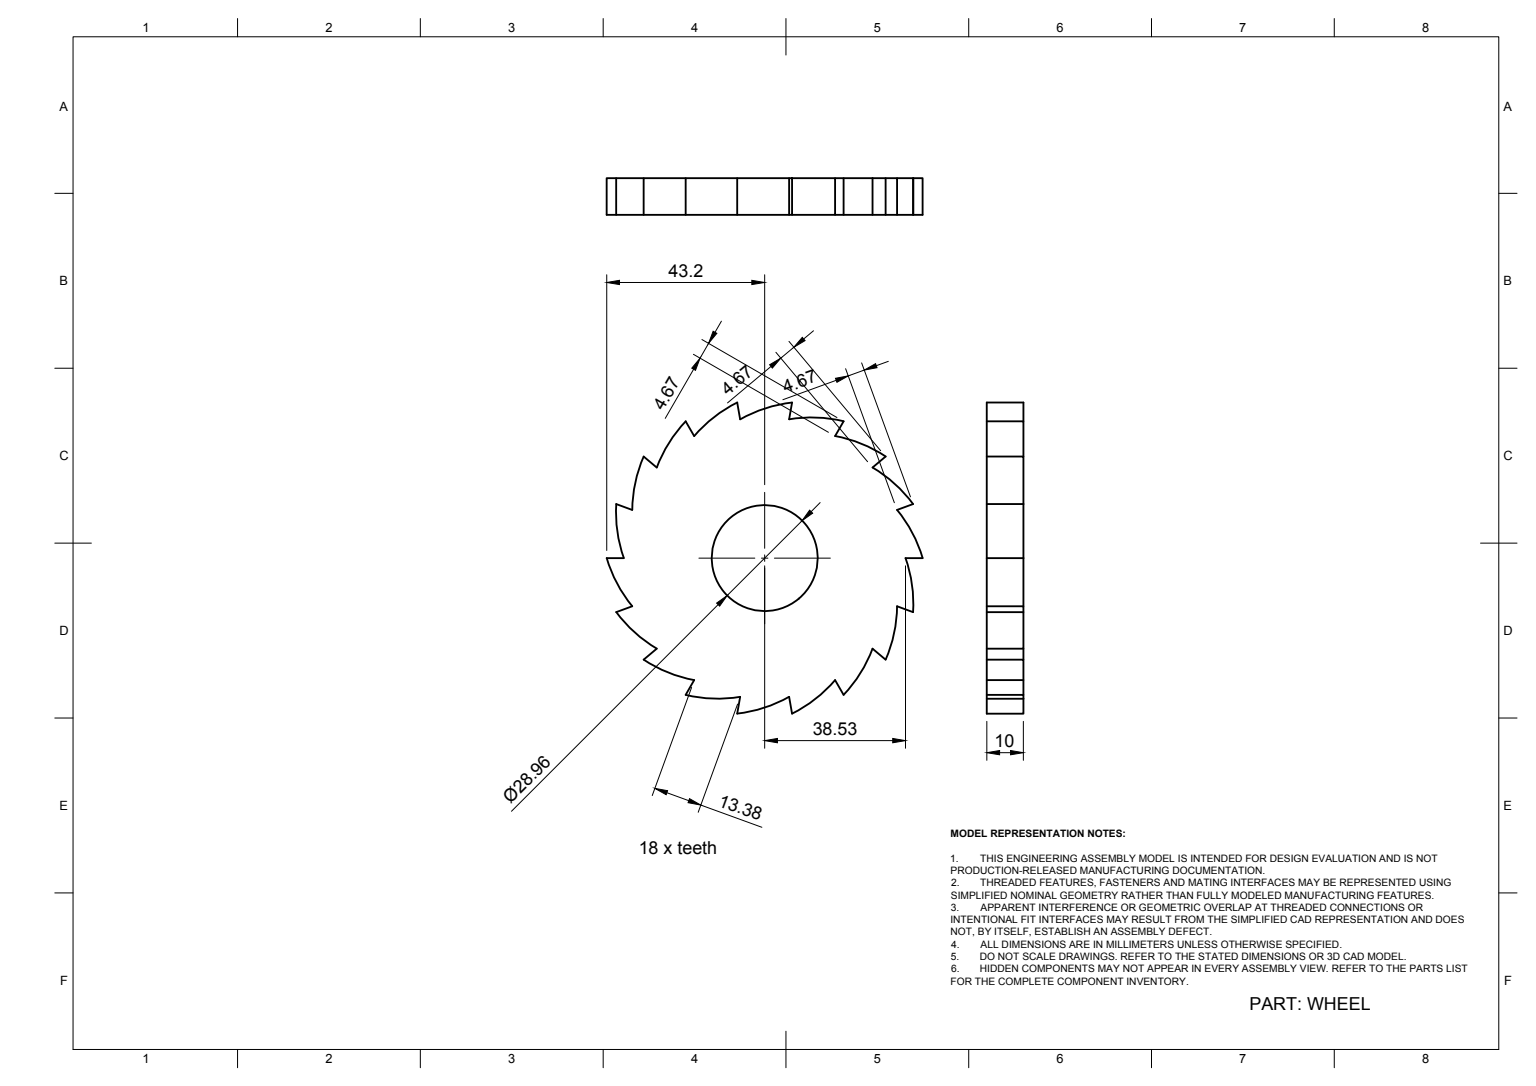
ISO-10303-21;
HEADER;
/* Generated by software containing ST-Developer
 * from STEP Tools, Inc. (www.steptools.com) 
 */

FILE_DESCRIPTION(
/* description */ (''),
/* implementation_level */ '2;1');

FILE_NAME(
/* name */ 'Wheel.step',
/* time_stamp */ '2026-09-20T22:38:01+06:00',
/* author */ (''),
/* organization */ (''),
/* preprocessor_version */ 'ST-DEVELOPER v20.2',
/* originating_system */ 'Autodesk Translation Framework v15.15.0.0',
/* authorisation */ '');

FILE_SCHEMA (('AUTOMOTIVE_DESIGN { 1 0 10303 214 3 1 1 }'));
ENDSEC;

DATA;
#10=MECHANICAL_DESIGN_GEOMETRIC_PRESENTATION_REPRESENTATION('',(#84),#4079);
#68=SHAPE_REPRESENTATION_RELATIONSHIP('SRR','None',#4111,#76);
#76=ADVANCED_BREP_SHAPE_REPRESENTATION('',(#92),#4071);
#84=STYLED_ITEM('',(#4160),#92);
#92=MANIFOLD_SOLID_BREP('Wheel',#1443);
#100=FACE_BOUND('',#285,.T.);
#101=FACE_BOUND('',#308,.T.);
#106=CIRCLE('',#1544,37.4987147312734);
#107=CIRCLE('',#1545,37.4987147312734);
#108=CIRCLE('',#1548,37.4987147312734);
#109=CIRCLE('',#1549,37.4987147312734);
#110=CIRCLE('',#1550,37.4987147312734);
#111=CIRCLE('',#1551,37.4987147312734);
#112=CIRCLE('',#1552,37.4987147312734);
#113=CIRCLE('',#1553,37.4987147312734);
#114=CIRCLE('',#1554,37.4987147312734);
#115=CIRCLE('',#1555,37.4987147312735);
#116=CIRCLE('',#1556,37.4987147312734);
#117=CIRCLE('',#1557,37.4987147312734);
#118=CIRCLE('',#1558,37.4987147312734);
#119=CIRCLE('',#1559,37.4987147312734);
#120=CIRCLE('',#1560,37.4987147312734);
#121=CIRCLE('',#1561,37.4987147312734);
#122=CIRCLE('',#1562,37.4987147312734);
#123=CIRCLE('',#1563,37.4987147312734);
#124=CIRCLE('',#1564,37.4987147312734);
#125=CIRCLE('',#1565,14.4819556358054);
#126=CIRCLE('',#1568,37.4987147312734);
#127=CIRCLE('',#1572,37.4987147312734);
#128=CIRCLE('',#1575,37.4987147312734);
#129=CIRCLE('',#1577,37.4987147312734);
#130=CIRCLE('',#1579,37.4987147312734);
#131=CIRCLE('',#1582,37.4987147312734);
#132=CIRCLE('',#1585,37.4987147312734);
#133=CIRCLE('',#1587,37.4987147312734);
#134=CIRCLE('',#1589,37.4987147312734);
#135=CIRCLE('',#1592,37.4987147312734);
#136=CIRCLE('',#1595,37.4987147312734);
#137=CIRCLE('',#1598,37.4987147312735);
#138=CIRCLE('',#1600,37.4987147312734);
#139=CIRCLE('',#1601,37.4987147312734);
#140=CIRCLE('',#1602,37.4987147312734);
#141=CIRCLE('',#1603,37.4987147312734);
#142=CIRCLE('',#1604,37.4987147312734);
#143=CIRCLE('',#1605,14.4819556358054);
#169=CYLINDRICAL_SURFACE('',#1543,37.4987147312734);
#170=CYLINDRICAL_SURFACE('',#1567,37.4987147312734);
#171=CYLINDRICAL_SURFACE('',#1571,37.4987147312734);
#172=CYLINDRICAL_SURFACE('',#1574,37.4987147312734);
#173=CYLINDRICAL_SURFACE('',#1576,37.4987147312734);
#174=CYLINDRICAL_SURFACE('',#1578,37.4987147312734);
#175=CYLINDRICAL_SURFACE('',#1581,37.4987147312734);
#176=CYLINDRICAL_SURFACE('',#1584,37.4987147312734);
#177=CYLINDRICAL_SURFACE('',#1586,37.4987147312734);
#178=CYLINDRICAL_SURFACE('',#1588,37.4987147312734);
#179=CYLINDRICAL_SURFACE('',#1591,37.4987147312734);
#180=CYLINDRICAL_SURFACE('',#1594,37.4987147312734);
#181=CYLINDRICAL_SURFACE('',#1597,37.4987147312735);
#182=CYLINDRICAL_SURFACE('',#1606,37.4987147312734);
#183=CYLINDRICAL_SURFACE('',#1608,37.4987147312734);
#184=CYLINDRICAL_SURFACE('',#1611,37.4987147312734);
#185=CYLINDRICAL_SURFACE('',#1613,37.4987147312734);
#186=CYLINDRICAL_SURFACE('',#1615,37.4987147312734);
#187=CYLINDRICAL_SURFACE('',#1618,14.4819556358054);
#197=FACE_OUTER_BOUND('',#281,.T.);
#198=FACE_OUTER_BOUND('',#282,.T.);
#199=FACE_OUTER_BOUND('',#283,.T.);
#200=FACE_OUTER_BOUND('',#284,.T.);
#201=FACE_OUTER_BOUND('',#286,.T.);
#202=FACE_OUTER_BOUND('',#287,.T.);
#203=FACE_OUTER_BOUND('',#288,.T.);
#204=FACE_OUTER_BOUND('',#289,.T.);
#205=FACE_OUTER_BOUND('',#290,.T.);
#206=FACE_OUTER_BOUND('',#291,.T.);
#207=FACE_OUTER_BOUND('',#292,.T.);
#208=FACE_OUTER_BOUND('',#293,.T.);
#209=FACE_OUTER_BOUND('',#294,.T.);
#210=FACE_OUTER_BOUND('',#295,.T.);
#211=FACE_OUTER_BOUND('',#296,.T.);
#212=FACE_OUTER_BOUND('',#297,.T.);
#213=FACE_OUTER_BOUND('',#298,.T.);
#214=FACE_OUTER_BOUND('',#299,.T.);
#215=FACE_OUTER_BOUND('',#300,.T.);
#216=FACE_OUTER_BOUND('',#301,.T.);
#217=FACE_OUTER_BOUND('',#302,.T.);
#218=FACE_OUTER_BOUND('',#303,.T.);
#219=FACE_OUTER_BOUND('',#304,.T.);
#220=FACE_OUTER_BOUND('',#305,.T.);
#221=FACE_OUTER_BOUND('',#306,.T.);
#222=FACE_OUTER_BOUND('',#307,.T.);
#223=FACE_OUTER_BOUND('',#309,.T.);
#224=FACE_OUTER_BOUND('',#310,.T.);
#225=FACE_OUTER_BOUND('',#311,.T.);
#226=FACE_OUTER_BOUND('',#312,.T.);
#227=FACE_OUTER_BOUND('',#313,.T.);
#228=FACE_OUTER_BOUND('',#314,.T.);
#229=FACE_OUTER_BOUND('',#315,.T.);
#230=FACE_OUTER_BOUND('',#316,.T.);
#231=FACE_OUTER_BOUND('',#317,.T.);
#232=FACE_OUTER_BOUND('',#318,.T.);
#233=FACE_OUTER_BOUND('',#319,.T.);
#234=FACE_OUTER_BOUND('',#320,.T.);
#235=FACE_OUTER_BOUND('',#321,.T.);
#281=EDGE_LOOP('',(#919,#920,#921,#922));
#282=EDGE_LOOP('',(#923,#924,#925,#926));
#283=EDGE_LOOP('',(#927,#928,#929,#930));
#284=EDGE_LOOP('',(#931,#932,#933,#934,#935,#936,#937,#938,#939,#940,#941,
#942,#943,#944,#945,#946,#947,#948,#949,#950,#951,#952,#953,#954,#955,#956,
#957,#958,#959,#960,#961,#962,#963,#964,#965,#966));
#285=EDGE_LOOP('',(#967));
#286=EDGE_LOOP('',(#968,#969,#970,#971));
#287=EDGE_LOOP('',(#972,#973,#974,#975));
#288=EDGE_LOOP('',(#976,#977,#978,#979));
#289=EDGE_LOOP('',(#980,#981,#982,#983));
#290=EDGE_LOOP('',(#984,#985,#986,#987));
#291=EDGE_LOOP('',(#988,#989,#990,#991));
#292=EDGE_LOOP('',(#992,#993,#994,#995));
#293=EDGE_LOOP('',(#996,#997,#998,#999));
#294=EDGE_LOOP('',(#1000,#1001,#1002,#1003));
#295=EDGE_LOOP('',(#1004,#1005,#1006,#1007));
#296=EDGE_LOOP('',(#1008,#1009,#1010,#1011));
#297=EDGE_LOOP('',(#1012,#1013,#1014,#1015));
#298=EDGE_LOOP('',(#1016,#1017,#1018,#1019));
#299=EDGE_LOOP('',(#1020,#1021,#1022,#1023));
#300=EDGE_LOOP('',(#1024,#1025,#1026,#1027));
#301=EDGE_LOOP('',(#1028,#1029,#1030,#1031));
#302=EDGE_LOOP('',(#1032,#1033,#1034,#1035));
#303=EDGE_LOOP('',(#1036,#1037,#1038,#1039));
#304=EDGE_LOOP('',(#1040,#1041,#1042,#1043));
#305=EDGE_LOOP('',(#1044,#1045,#1046,#1047));
#306=EDGE_LOOP('',(#1048,#1049,#1050,#1051));
#307=EDGE_LOOP('',(#1052,#1053,#1054,#1055,#1056,#1057,#1058,#1059,#1060,
#1061,#1062,#1063,#1064,#1065,#1066,#1067,#1068,#1069,#1070,#1071,#1072,
#1073,#1074,#1075,#1076,#1077,#1078,#1079,#1080,#1081,#1082,#1083,#1084,
#1085,#1086,#1087));
#308=EDGE_LOOP('',(#1088));
#309=EDGE_LOOP('',(#1089,#1090,#1091,#1092));
#310=EDGE_LOOP('',(#1093,#1094,#1095,#1096));
#311=EDGE_LOOP('',(#1097,#1098,#1099,#1100));
#312=EDGE_LOOP('',(#1101,#1102,#1103,#1104));
#313=EDGE_LOOP('',(#1105,#1106,#1107,#1108));
#314=EDGE_LOOP('',(#1109,#1110,#1111,#1112));
#315=EDGE_LOOP('',(#1113,#1114,#1115,#1116));
#316=EDGE_LOOP('',(#1117,#1118,#1119,#1120));
#317=EDGE_LOOP('',(#1121,#1122,#1123,#1124));
#318=EDGE_LOOP('',(#1125,#1126,#1127,#1128));
#319=EDGE_LOOP('',(#1129,#1130,#1131,#1132));
#320=EDGE_LOOP('',(#1133,#1134,#1135,#1136));
#321=EDGE_LOOP('',(#1137,#1138,#1139,#1140));
#371=LINE('',#2132,#484);
#372=LINE('',#2134,#485);
#373=LINE('',#2136,#486);
#374=LINE('',#2137,#487);
#375=LINE('',#2141,#488);
#376=LINE('',#2146,#489);
#377=LINE('',#2148,#490);
#378=LINE('',#2149,#491);
#379=LINE('',#2154,#492);
#380=LINE('',#2158,#493);
#381=LINE('',#2162,#494);
#382=LINE('',#2166,#495);
#383=LINE('',#2170,#496);
#384=LINE('',#2174,#497);
#385=LINE('',#2178,#498);
#386=LINE('',#2182,#499);
#387=LINE('',#2186,#500);
#388=LINE('',#2190,#501);
#389=LINE('',#2194,#502);
#390=LINE('',#2198,#503);
#391=LINE('',#2202,#504);
#392=LINE('',#2206,#505);
#393=LINE('',#2210,#506);
#394=LINE('',#2214,#507);
#395=LINE('',#2220,#508);
#396=LINE('',#2222,#509);
#397=LINE('',#2223,#510);
#398=LINE('',#2226,#511);
#399=LINE('',#2230,#512);
#400=LINE('',#2231,#513);
#401=LINE('',#2234,#514);
#402=LINE('',#2236,#515);
#403=LINE('',#2237,#516);
#404=LINE('',#2240,#517);
#405=LINE('',#2244,#518);
#406=LINE('',#2245,#519);
#407=LINE('',#2250,#520);
#408=LINE('',#2255,#521);
#409=LINE('',#2257,#522);
#410=LINE('',#2260,#523);
#411=LINE('',#2263,#524);
#412=LINE('',#2266,#525);
#413=LINE('',#2267,#526);
#414=LINE('',#2271,#527);
#415=LINE('',#2274,#528);
#416=LINE('',#2279,#529);
#417=LINE('',#2281,#530);
#418=LINE('',#2284,#531);
#419=LINE('',#2287,#532);
#420=LINE('',#2290,#533);
#421=LINE('',#2291,#534);
#422=LINE('',#2294,#535);
#423=LINE('',#2297,#536);
#424=LINE('',#2300,#537);
#425=LINE('',#2301,#538);
#426=LINE('',#2305,#539);
#427=LINE('',#2308,#540);
#428=LINE('',#2312,#541);
#429=LINE('',#2316,#542);
#430=LINE('',#2319,#543);
#431=LINE('',#2321,#544);
#432=LINE('',#2325,#545);
#433=LINE('',#2327,#546);
#434=LINE('',#2331,#547);
#435=LINE('',#2332,#548);
#436=LINE('',#2335,#549);
#437=LINE('',#2338,#550);
#438=LINE('',#2339,#551);
#439=LINE('',#2341,#552);
#440=LINE('',#2344,#553);
#441=LINE('',#2345,#554);
#442=LINE('',#2348,#555);
#443=LINE('',#2352,#556);
#484=VECTOR('',#1704,10.);
#485=VECTOR('',#1705,10.);
#486=VECTOR('',#1706,10.);
#487=VECTOR('',#1707,10.);
#488=VECTOR('',#1710,10.);
#489=VECTOR('',#1717,10.);
#490=VECTOR('',#1718,10.);
#491=VECTOR('',#1719,10.);
#492=VECTOR('',#1724,10.);
#493=VECTOR('',#1727,10.);
#494=VECTOR('',#1730,10.);
#495=VECTOR('',#1733,10.);
#496=VECTOR('',#1736,10.);
#497=VECTOR('',#1739,10.);
#498=VECTOR('',#1742,10.);
#499=VECTOR('',#1745,10.);
#500=VECTOR('',#1748,10.);
#501=VECTOR('',#1751,10.);
#502=VECTOR('',#1754,10.);
#503=VECTOR('',#1757,10.);
#504=VECTOR('',#1760,10.);
#505=VECTOR('',#1763,10.);
#506=VECTOR('',#1766,10.);
#507=VECTOR('',#1769,10.);
#508=VECTOR('',#1776,10.);
#509=VECTOR('',#1777,10.);
#510=VECTOR('',#1778,10.);
#511=VECTOR('',#1781,10.);
#512=VECTOR('',#1786,10.);
#513=VECTOR('',#1787,10.);
#514=VECTOR('',#1790,10.);
#515=VECTOR('',#1791,10.);
#516=VECTOR('',#1792,10.);
#517=VECTOR('',#1795,10.);
#518=VECTOR('',#1800,10.);
#519=VECTOR('',#1801,10.);
#520=VECTOR('',#1808,10.);
#521=VECTOR('',#1815,10.);
#522=VECTOR('',#1818,10.);
#523=VECTOR('',#1821,10.);
#524=VECTOR('',#1824,10.);
#525=VECTOR('',#1827,10.);
#526=VECTOR('',#1828,10.);
#527=VECTOR('',#1833,10.);
#528=VECTOR('',#1836,10.);
#529=VECTOR('',#1843,10.);
#530=VECTOR('',#1846,10.);
#531=VECTOR('',#1849,10.);
#532=VECTOR('',#1852,10.);
#533=VECTOR('',#1855,10.);
#534=VECTOR('',#1856,10.);
#535=VECTOR('',#1859,10.);
#536=VECTOR('',#1862,10.);
#537=VECTOR('',#1865,10.);
#538=VECTOR('',#1866,10.);
#539=VECTOR('',#1871,10.);
#540=VECTOR('',#1874,10.);
#541=VECTOR('',#1877,10.);
#542=VECTOR('',#1880,10.);
#543=VECTOR('',#1883,10.);
#544=VECTOR('',#1884,10.);
#545=VECTOR('',#1887,10.);
#546=VECTOR('',#1890,10.);
#547=VECTOR('',#1895,10.);
#548=VECTOR('',#1896,10.);
#549=VECTOR('',#1901,10.);
#550=VECTOR('',#1906,10.);
#551=VECTOR('',#1907,10.);
#552=VECTOR('',#1910,10.);
#553=VECTOR('',#1915,10.);
#554=VECTOR('',#1916,10.);
#555=VECTOR('',#1921,10.);
#556=VECTOR('',#1928,14.4819556358054);
#597=VERTEX_POINT('',#2130);
#598=VERTEX_POINT('',#2131);
#599=VERTEX_POINT('',#2133);
#600=VERTEX_POINT('',#2135);
#601=VERTEX_POINT('',#2139);
#602=VERTEX_POINT('',#2140);
#603=VERTEX_POINT('',#2145);
#604=VERTEX_POINT('',#2147);
#605=VERTEX_POINT('',#2151);
#606=VERTEX_POINT('',#2153);
#607=VERTEX_POINT('',#2155);
#608=VERTEX_POINT('',#2157);
#609=VERTEX_POINT('',#2159);
#610=VERTEX_POINT('',#2161);
#611=VERTEX_POINT('',#2163);
#612=VERTEX_POINT('',#2165);
#613=VERTEX_POINT('',#2167);
#614=VERTEX_POINT('',#2169);
#615=VERTEX_POINT('',#2171);
#616=VERTEX_POINT('',#2173);
#617=VERTEX_POINT('',#2175);
#618=VERTEX_POINT('',#2177);
#619=VERTEX_POINT('',#2179);
#620=VERTEX_POINT('',#2181);
#621=VERTEX_POINT('',#2183);
#622=VERTEX_POINT('',#2185);
#623=VERTEX_POINT('',#2187);
#624=VERTEX_POINT('',#2189);
#625=VERTEX_POINT('',#2191);
#626=VERTEX_POINT('',#2193);
#627=VERTEX_POINT('',#2195);
#628=VERTEX_POINT('',#2197);
#629=VERTEX_POINT('',#2199);
#630=VERTEX_POINT('',#2201);
#631=VERTEX_POINT('',#2203);
#632=VERTEX_POINT('',#2205);
#633=VERTEX_POINT('',#2207);
#634=VERTEX_POINT('',#2209);
#635=VERTEX_POINT('',#2211);
#636=VERTEX_POINT('',#2213);
#637=VERTEX_POINT('',#2216);
#638=VERTEX_POINT('',#2219);
#639=VERTEX_POINT('',#2221);
#640=VERTEX_POINT('',#2225);
#641=VERTEX_POINT('',#2229);
#642=VERTEX_POINT('',#2233);
#643=VERTEX_POINT('',#2235);
#644=VERTEX_POINT('',#2239);
#645=VERTEX_POINT('',#2243);
#646=VERTEX_POINT('',#2249);
#647=VERTEX_POINT('',#2253);
#648=VERTEX_POINT('',#2259);
#649=VERTEX_POINT('',#2261);
#650=VERTEX_POINT('',#2265);
#651=VERTEX_POINT('',#2269);
#652=VERTEX_POINT('',#2273);
#653=VERTEX_POINT('',#2277);
#654=VERTEX_POINT('',#2283);
#655=VERTEX_POINT('',#2285);
#656=VERTEX_POINT('',#2289);
#657=VERTEX_POINT('',#2293);
#658=VERTEX_POINT('',#2295);
#659=VERTEX_POINT('',#2299);
#660=VERTEX_POINT('',#2303);
#661=VERTEX_POINT('',#2307);
#662=VERTEX_POINT('',#2309);
#663=VERTEX_POINT('',#2311);
#664=VERTEX_POINT('',#2313);
#665=VERTEX_POINT('',#2315);
#666=VERTEX_POINT('',#2317);
#667=VERTEX_POINT('',#2320);
#668=VERTEX_POINT('',#2322);
#669=VERTEX_POINT('',#2324);
#670=VERTEX_POINT('',#2328);
#724=EDGE_CURVE('',#597,#598,#371,.T.);
#725=EDGE_CURVE('',#597,#599,#372,.T.);
#726=EDGE_CURVE('',#599,#600,#373,.T.);
#727=EDGE_CURVE('',#598,#600,#374,.T.);
#728=EDGE_CURVE('',#601,#602,#375,.T.);
#729=EDGE_CURVE('',#600,#601,#106,.T.);
#730=EDGE_CURVE('',#602,#599,#107,.T.);
#731=EDGE_CURVE('',#602,#603,#376,.T.);
#732=EDGE_CURVE('',#603,#604,#377,.T.);
#733=EDGE_CURVE('',#601,#604,#378,.T.);
#734=EDGE_CURVE('',#597,#605,#108,.T.);
#735=EDGE_CURVE('',#606,#605,#379,.T.);
#736=EDGE_CURVE('',#606,#607,#109,.T.);
#737=EDGE_CURVE('',#608,#607,#380,.T.);
#738=EDGE_CURVE('',#608,#609,#110,.T.);
#739=EDGE_CURVE('',#610,#609,#381,.T.);
#740=EDGE_CURVE('',#610,#611,#111,.T.);
#741=EDGE_CURVE('',#612,#611,#382,.T.);
#742=EDGE_CURVE('',#612,#613,#112,.T.);
#743=EDGE_CURVE('',#614,#613,#383,.T.);
#744=EDGE_CURVE('',#614,#615,#113,.T.);
#745=EDGE_CURVE('',#616,#615,#384,.T.);
#746=EDGE_CURVE('',#616,#617,#114,.T.);
#747=EDGE_CURVE('',#618,#617,#385,.T.);
#748=EDGE_CURVE('',#618,#619,#115,.T.);
#749=EDGE_CURVE('',#620,#619,#386,.T.);
#750=EDGE_CURVE('',#620,#621,#116,.T.);
#751=EDGE_CURVE('',#622,#621,#387,.T.);
#752=EDGE_CURVE('',#622,#623,#117,.T.);
#753=EDGE_CURVE('',#624,#623,#388,.T.);
#754=EDGE_CURVE('',#624,#625,#118,.T.);
#755=EDGE_CURVE('',#626,#625,#389,.T.);
#756=EDGE_CURVE('',#626,#627,#119,.T.);
#757=EDGE_CURVE('',#628,#627,#390,.T.);
#758=EDGE_CURVE('',#628,#629,#120,.T.);
#759=EDGE_CURVE('',#630,#629,#391,.T.);
#760=EDGE_CURVE('',#630,#631,#121,.T.);
#761=EDGE_CURVE('',#632,#631,#392,.T.);
#762=EDGE_CURVE('',#632,#633,#122,.T.);
#763=EDGE_CURVE('',#634,#633,#393,.T.);
#764=EDGE_CURVE('',#634,#635,#123,.T.);
#765=EDGE_CURVE('',#636,#635,#394,.T.);
#766=EDGE_CURVE('',#636,#603,#124,.T.);
#767=EDGE_CURVE('',#637,#637,#125,.T.);
#768=EDGE_CURVE('',#636,#638,#395,.T.);
#769=EDGE_CURVE('',#635,#639,#396,.T.);
#770=EDGE_CURVE('',#638,#639,#397,.T.);
#771=EDGE_CURVE('',#640,#634,#398,.T.);
#772=EDGE_CURVE('',#639,#640,#126,.T.);
#773=EDGE_CURVE('',#633,#641,#399,.T.);
#774=EDGE_CURVE('',#640,#641,#400,.T.);
#775=EDGE_CURVE('',#630,#642,#401,.T.);
#776=EDGE_CURVE('',#629,#643,#402,.T.);
#777=EDGE_CURVE('',#642,#643,#403,.T.);
#778=EDGE_CURVE('',#644,#628,#404,.T.);
#779=EDGE_CURVE('',#643,#644,#127,.T.);
#780=EDGE_CURVE('',#627,#645,#405,.T.);
#781=EDGE_CURVE('',#644,#645,#406,.T.);
#782=EDGE_CURVE('',#604,#638,#128,.T.);
#783=EDGE_CURVE('',#646,#632,#407,.T.);
#784=EDGE_CURVE('',#641,#646,#129,.T.);
#785=EDGE_CURVE('',#647,#642,#130,.T.);
#786=EDGE_CURVE('',#631,#647,#408,.T.);
#787=EDGE_CURVE('',#646,#647,#409,.T.);
#788=EDGE_CURVE('',#648,#606,#410,.T.);
#789=EDGE_CURVE('',#649,#648,#131,.T.);
#790=EDGE_CURVE('',#607,#649,#411,.T.);
#791=EDGE_CURVE('',#608,#650,#412,.T.);
#792=EDGE_CURVE('',#650,#649,#413,.T.);
#793=EDGE_CURVE('',#651,#650,#132,.T.);
#794=EDGE_CURVE('',#609,#651,#414,.T.);
#795=EDGE_CURVE('',#652,#626,#415,.T.);
#796=EDGE_CURVE('',#645,#652,#133,.T.);
#797=EDGE_CURVE('',#653,#598,#134,.T.);
#798=EDGE_CURVE('',#605,#653,#416,.T.);
#799=EDGE_CURVE('',#648,#653,#417,.T.);
#800=EDGE_CURVE('',#654,#610,#418,.T.);
#801=EDGE_CURVE('',#655,#654,#135,.T.);
#802=EDGE_CURVE('',#611,#655,#419,.T.);
#803=EDGE_CURVE('',#612,#656,#420,.T.);
#804=EDGE_CURVE('',#656,#655,#421,.T.);
#805=EDGE_CURVE('',#657,#616,#422,.T.);
#806=EDGE_CURVE('',#658,#657,#136,.T.);
#807=EDGE_CURVE('',#617,#658,#423,.T.);
#808=EDGE_CURVE('',#618,#659,#424,.T.);
#809=EDGE_CURVE('',#659,#658,#425,.T.);
#810=EDGE_CURVE('',#660,#659,#137,.T.);
#811=EDGE_CURVE('',#619,#660,#426,.T.);
#812=EDGE_CURVE('',#652,#661,#427,.T.);
#813=EDGE_CURVE('',#661,#662,#138,.T.);
#814=EDGE_CURVE('',#662,#663,#428,.T.);
#815=EDGE_CURVE('',#663,#664,#139,.T.);
#816=EDGE_CURVE('',#664,#665,#429,.T.);
#817=EDGE_CURVE('',#665,#666,#140,.T.);
#818=EDGE_CURVE('',#666,#660,#430,.T.);
#819=EDGE_CURVE('',#657,#667,#431,.T.);
#820=EDGE_CURVE('',#667,#668,#141,.T.);
#821=EDGE_CURVE('',#668,#669,#432,.T.);
#822=EDGE_CURVE('',#669,#656,#142,.T.);
#823=EDGE_CURVE('',#654,#651,#433,.T.);
#824=EDGE_CURVE('',#670,#670,#143,.T.);
#825=EDGE_CURVE('',#668,#614,#434,.T.);
#826=EDGE_CURVE('',#615,#667,#435,.T.);
#827=EDGE_CURVE('',#613,#669,#436,.T.);
#828=EDGE_CURVE('',#622,#664,#437,.T.);
#829=EDGE_CURVE('',#621,#665,#438,.T.);
#830=EDGE_CURVE('',#666,#620,#439,.T.);
#831=EDGE_CURVE('',#662,#624,#440,.T.);
#832=EDGE_CURVE('',#625,#661,#441,.T.);
#833=EDGE_CURVE('',#623,#663,#442,.T.);
#834=EDGE_CURVE('',#670,#637,#443,.T.);
#919=ORIENTED_EDGE('',*,*,#724,.F.);
#920=ORIENTED_EDGE('',*,*,#725,.T.);
#921=ORIENTED_EDGE('',*,*,#726,.T.);
#922=ORIENTED_EDGE('',*,*,#727,.F.);
#923=ORIENTED_EDGE('',*,*,#728,.F.);
#924=ORIENTED_EDGE('',*,*,#729,.F.);
#925=ORIENTED_EDGE('',*,*,#726,.F.);
#926=ORIENTED_EDGE('',*,*,#730,.F.);
#927=ORIENTED_EDGE('',*,*,#728,.T.);
#928=ORIENTED_EDGE('',*,*,#731,.T.);
#929=ORIENTED_EDGE('',*,*,#732,.T.);
#930=ORIENTED_EDGE('',*,*,#733,.F.);
#931=ORIENTED_EDGE('',*,*,#730,.T.);
#932=ORIENTED_EDGE('',*,*,#725,.F.);
#933=ORIENTED_EDGE('',*,*,#734,.T.);
#934=ORIENTED_EDGE('',*,*,#735,.F.);
#935=ORIENTED_EDGE('',*,*,#736,.T.);
#936=ORIENTED_EDGE('',*,*,#737,.F.);
#937=ORIENTED_EDGE('',*,*,#738,.T.);
#938=ORIENTED_EDGE('',*,*,#739,.F.);
#939=ORIENTED_EDGE('',*,*,#740,.T.);
#940=ORIENTED_EDGE('',*,*,#741,.F.);
#941=ORIENTED_EDGE('',*,*,#742,.T.);
#942=ORIENTED_EDGE('',*,*,#743,.F.);
#943=ORIENTED_EDGE('',*,*,#744,.T.);
#944=ORIENTED_EDGE('',*,*,#745,.F.);
#945=ORIENTED_EDGE('',*,*,#746,.T.);
#946=ORIENTED_EDGE('',*,*,#747,.F.);
#947=ORIENTED_EDGE('',*,*,#748,.T.);
#948=ORIENTED_EDGE('',*,*,#749,.F.);
#949=ORIENTED_EDGE('',*,*,#750,.T.);
#950=ORIENTED_EDGE('',*,*,#751,.F.);
#951=ORIENTED_EDGE('',*,*,#752,.T.);
#952=ORIENTED_EDGE('',*,*,#753,.F.);
#953=ORIENTED_EDGE('',*,*,#754,.T.);
#954=ORIENTED_EDGE('',*,*,#755,.F.);
#955=ORIENTED_EDGE('',*,*,#756,.T.);
#956=ORIENTED_EDGE('',*,*,#757,.F.);
#957=ORIENTED_EDGE('',*,*,#758,.T.);
#958=ORIENTED_EDGE('',*,*,#759,.F.);
#959=ORIENTED_EDGE('',*,*,#760,.T.);
#960=ORIENTED_EDGE('',*,*,#761,.F.);
#961=ORIENTED_EDGE('',*,*,#762,.T.);
#962=ORIENTED_EDGE('',*,*,#763,.F.);
#963=ORIENTED_EDGE('',*,*,#764,.T.);
#964=ORIENTED_EDGE('',*,*,#765,.F.);
#965=ORIENTED_EDGE('',*,*,#766,.T.);
#966=ORIENTED_EDGE('',*,*,#731,.F.);
#967=ORIENTED_EDGE('',*,*,#767,.T.);
#968=ORIENTED_EDGE('',*,*,#768,.F.);
#969=ORIENTED_EDGE('',*,*,#765,.T.);
#970=ORIENTED_EDGE('',*,*,#769,.T.);
#971=ORIENTED_EDGE('',*,*,#770,.F.);
#972=ORIENTED_EDGE('',*,*,#771,.F.);
#973=ORIENTED_EDGE('',*,*,#772,.F.);
#974=ORIENTED_EDGE('',*,*,#769,.F.);
#975=ORIENTED_EDGE('',*,*,#764,.F.);
#976=ORIENTED_EDGE('',*,*,#771,.T.);
#977=ORIENTED_EDGE('',*,*,#763,.T.);
#978=ORIENTED_EDGE('',*,*,#773,.T.);
#979=ORIENTED_EDGE('',*,*,#774,.F.);
#980=ORIENTED_EDGE('',*,*,#775,.F.);
#981=ORIENTED_EDGE('',*,*,#759,.T.);
#982=ORIENTED_EDGE('',*,*,#776,.T.);
#983=ORIENTED_EDGE('',*,*,#777,.F.);
#984=ORIENTED_EDGE('',*,*,#778,.F.);
#985=ORIENTED_EDGE('',*,*,#779,.F.);
#986=ORIENTED_EDGE('',*,*,#776,.F.);
#987=ORIENTED_EDGE('',*,*,#758,.F.);
#988=ORIENTED_EDGE('',*,*,#778,.T.);
#989=ORIENTED_EDGE('',*,*,#757,.T.);
#990=ORIENTED_EDGE('',*,*,#780,.T.);
#991=ORIENTED_EDGE('',*,*,#781,.F.);
#992=ORIENTED_EDGE('',*,*,#768,.T.);
#993=ORIENTED_EDGE('',*,*,#782,.F.);
#994=ORIENTED_EDGE('',*,*,#732,.F.);
#995=ORIENTED_EDGE('',*,*,#766,.F.);
#996=ORIENTED_EDGE('',*,*,#783,.F.);
#997=ORIENTED_EDGE('',*,*,#784,.F.);
#998=ORIENTED_EDGE('',*,*,#773,.F.);
#999=ORIENTED_EDGE('',*,*,#762,.F.);
#1000=ORIENTED_EDGE('',*,*,#775,.T.);
#1001=ORIENTED_EDGE('',*,*,#785,.F.);
#1002=ORIENTED_EDGE('',*,*,#786,.F.);
#1003=ORIENTED_EDGE('',*,*,#760,.F.);
#1004=ORIENTED_EDGE('',*,*,#783,.T.);
#1005=ORIENTED_EDGE('',*,*,#761,.T.);
#1006=ORIENTED_EDGE('',*,*,#786,.T.);
#1007=ORIENTED_EDGE('',*,*,#787,.F.);
#1008=ORIENTED_EDGE('',*,*,#788,.F.);
#1009=ORIENTED_EDGE('',*,*,#789,.F.);
#1010=ORIENTED_EDGE('',*,*,#790,.F.);
#1011=ORIENTED_EDGE('',*,*,#736,.F.);
#1012=ORIENTED_EDGE('',*,*,#791,.F.);
#1013=ORIENTED_EDGE('',*,*,#737,.T.);
#1014=ORIENTED_EDGE('',*,*,#790,.T.);
#1015=ORIENTED_EDGE('',*,*,#792,.F.);
#1016=ORIENTED_EDGE('',*,*,#791,.T.);
#1017=ORIENTED_EDGE('',*,*,#793,.F.);
#1018=ORIENTED_EDGE('',*,*,#794,.F.);
#1019=ORIENTED_EDGE('',*,*,#738,.F.);
#1020=ORIENTED_EDGE('',*,*,#795,.F.);
#1021=ORIENTED_EDGE('',*,*,#796,.F.);
#1022=ORIENTED_EDGE('',*,*,#780,.F.);
#1023=ORIENTED_EDGE('',*,*,#756,.F.);
#1024=ORIENTED_EDGE('',*,*,#724,.T.);
#1025=ORIENTED_EDGE('',*,*,#797,.F.);
#1026=ORIENTED_EDGE('',*,*,#798,.F.);
#1027=ORIENTED_EDGE('',*,*,#734,.F.);
#1028=ORIENTED_EDGE('',*,*,#788,.T.);
#1029=ORIENTED_EDGE('',*,*,#735,.T.);
#1030=ORIENTED_EDGE('',*,*,#798,.T.);
#1031=ORIENTED_EDGE('',*,*,#799,.F.);
#1032=ORIENTED_EDGE('',*,*,#800,.F.);
#1033=ORIENTED_EDGE('',*,*,#801,.F.);
#1034=ORIENTED_EDGE('',*,*,#802,.F.);
#1035=ORIENTED_EDGE('',*,*,#740,.F.);
#1036=ORIENTED_EDGE('',*,*,#803,.F.);
#1037=ORIENTED_EDGE('',*,*,#741,.T.);
#1038=ORIENTED_EDGE('',*,*,#802,.T.);
#1039=ORIENTED_EDGE('',*,*,#804,.F.);
#1040=ORIENTED_EDGE('',*,*,#805,.F.);
#1041=ORIENTED_EDGE('',*,*,#806,.F.);
#1042=ORIENTED_EDGE('',*,*,#807,.F.);
#1043=ORIENTED_EDGE('',*,*,#746,.F.);
#1044=ORIENTED_EDGE('',*,*,#808,.F.);
#1045=ORIENTED_EDGE('',*,*,#747,.T.);
#1046=ORIENTED_EDGE('',*,*,#807,.T.);
#1047=ORIENTED_EDGE('',*,*,#809,.F.);
#1048=ORIENTED_EDGE('',*,*,#808,.T.);
#1049=ORIENTED_EDGE('',*,*,#810,.F.);
#1050=ORIENTED_EDGE('',*,*,#811,.F.);
#1051=ORIENTED_EDGE('',*,*,#748,.F.);
#1052=ORIENTED_EDGE('',*,*,#733,.T.);
#1053=ORIENTED_EDGE('',*,*,#782,.T.);
#1054=ORIENTED_EDGE('',*,*,#770,.T.);
#1055=ORIENTED_EDGE('',*,*,#772,.T.);
#1056=ORIENTED_EDGE('',*,*,#774,.T.);
#1057=ORIENTED_EDGE('',*,*,#784,.T.);
#1058=ORIENTED_EDGE('',*,*,#787,.T.);
#1059=ORIENTED_EDGE('',*,*,#785,.T.);
#1060=ORIENTED_EDGE('',*,*,#777,.T.);
#1061=ORIENTED_EDGE('',*,*,#779,.T.);
#1062=ORIENTED_EDGE('',*,*,#781,.T.);
#1063=ORIENTED_EDGE('',*,*,#796,.T.);
#1064=ORIENTED_EDGE('',*,*,#812,.T.);
#1065=ORIENTED_EDGE('',*,*,#813,.T.);
#1066=ORIENTED_EDGE('',*,*,#814,.T.);
#1067=ORIENTED_EDGE('',*,*,#815,.T.);
#1068=ORIENTED_EDGE('',*,*,#816,.T.);
#1069=ORIENTED_EDGE('',*,*,#817,.T.);
#1070=ORIENTED_EDGE('',*,*,#818,.T.);
#1071=ORIENTED_EDGE('',*,*,#810,.T.);
#1072=ORIENTED_EDGE('',*,*,#809,.T.);
#1073=ORIENTED_EDGE('',*,*,#806,.T.);
#1074=ORIENTED_EDGE('',*,*,#819,.T.);
#1075=ORIENTED_EDGE('',*,*,#820,.T.);
#1076=ORIENTED_EDGE('',*,*,#821,.T.);
#1077=ORIENTED_EDGE('',*,*,#822,.T.);
#1078=ORIENTED_EDGE('',*,*,#804,.T.);
#1079=ORIENTED_EDGE('',*,*,#801,.T.);
#1080=ORIENTED_EDGE('',*,*,#823,.T.);
#1081=ORIENTED_EDGE('',*,*,#793,.T.);
#1082=ORIENTED_EDGE('',*,*,#792,.T.);
#1083=ORIENTED_EDGE('',*,*,#789,.T.);
#1084=ORIENTED_EDGE('',*,*,#799,.T.);
#1085=ORIENTED_EDGE('',*,*,#797,.T.);
#1086=ORIENTED_EDGE('',*,*,#727,.T.);
#1087=ORIENTED_EDGE('',*,*,#729,.T.);
#1088=ORIENTED_EDGE('',*,*,#824,.T.);
#1089=ORIENTED_EDGE('',*,*,#825,.F.);
#1090=ORIENTED_EDGE('',*,*,#820,.F.);
#1091=ORIENTED_EDGE('',*,*,#826,.F.);
#1092=ORIENTED_EDGE('',*,*,#744,.F.);
#1093=ORIENTED_EDGE('',*,*,#805,.T.);
#1094=ORIENTED_EDGE('',*,*,#745,.T.);
#1095=ORIENTED_EDGE('',*,*,#826,.T.);
#1096=ORIENTED_EDGE('',*,*,#819,.F.);
#1097=ORIENTED_EDGE('',*,*,#803,.T.);
#1098=ORIENTED_EDGE('',*,*,#822,.F.);
#1099=ORIENTED_EDGE('',*,*,#827,.F.);
#1100=ORIENTED_EDGE('',*,*,#742,.F.);
#1101=ORIENTED_EDGE('',*,*,#825,.T.);
#1102=ORIENTED_EDGE('',*,*,#743,.T.);
#1103=ORIENTED_EDGE('',*,*,#827,.T.);
#1104=ORIENTED_EDGE('',*,*,#821,.F.);
#1105=ORIENTED_EDGE('',*,*,#828,.F.);
#1106=ORIENTED_EDGE('',*,*,#751,.T.);
#1107=ORIENTED_EDGE('',*,*,#829,.T.);
#1108=ORIENTED_EDGE('',*,*,#816,.F.);
#1109=ORIENTED_EDGE('',*,*,#830,.F.);
#1110=ORIENTED_EDGE('',*,*,#817,.F.);
#1111=ORIENTED_EDGE('',*,*,#829,.F.);
#1112=ORIENTED_EDGE('',*,*,#750,.F.);
#1113=ORIENTED_EDGE('',*,*,#830,.T.);
#1114=ORIENTED_EDGE('',*,*,#749,.T.);
#1115=ORIENTED_EDGE('',*,*,#811,.T.);
#1116=ORIENTED_EDGE('',*,*,#818,.F.);
#1117=ORIENTED_EDGE('',*,*,#831,.F.);
#1118=ORIENTED_EDGE('',*,*,#813,.F.);
#1119=ORIENTED_EDGE('',*,*,#832,.F.);
#1120=ORIENTED_EDGE('',*,*,#754,.F.);
#1121=ORIENTED_EDGE('',*,*,#795,.T.);
#1122=ORIENTED_EDGE('',*,*,#755,.T.);
#1123=ORIENTED_EDGE('',*,*,#832,.T.);
#1124=ORIENTED_EDGE('',*,*,#812,.F.);
#1125=ORIENTED_EDGE('',*,*,#828,.T.);
#1126=ORIENTED_EDGE('',*,*,#815,.F.);
#1127=ORIENTED_EDGE('',*,*,#833,.F.);
#1128=ORIENTED_EDGE('',*,*,#752,.F.);
#1129=ORIENTED_EDGE('',*,*,#831,.T.);
#1130=ORIENTED_EDGE('',*,*,#753,.T.);
#1131=ORIENTED_EDGE('',*,*,#833,.T.);
#1132=ORIENTED_EDGE('',*,*,#814,.F.);
#1133=ORIENTED_EDGE('',*,*,#800,.T.);
#1134=ORIENTED_EDGE('',*,*,#739,.T.);
#1135=ORIENTED_EDGE('',*,*,#794,.T.);
#1136=ORIENTED_EDGE('',*,*,#823,.F.);
#1137=ORIENTED_EDGE('',*,*,#824,.F.);
#1138=ORIENTED_EDGE('',*,*,#834,.T.);
#1139=ORIENTED_EDGE('',*,*,#767,.F.);
#1140=ORIENTED_EDGE('',*,*,#834,.F.);
#1309=PLANE('',#1542);
#1310=PLANE('',#1546);
#1311=PLANE('',#1547);
#1312=PLANE('',#1566);
#1313=PLANE('',#1569);
#1314=PLANE('',#1570);
#1315=PLANE('',#1573);
#1316=PLANE('',#1580);
#1317=PLANE('',#1583);
#1318=PLANE('',#1590);
#1319=PLANE('',#1593);
#1320=PLANE('',#1596);
#1321=PLANE('',#1599);
#1322=PLANE('',#1607);
#1323=PLANE('',#1609);
#1324=PLANE('',#1610);
#1325=PLANE('',#1612);
#1326=PLANE('',#1614);
#1327=PLANE('',#1616);
#1328=PLANE('',#1617);
#1359=ADVANCED_FACE('',(#197),#1309,.T.);
#1360=ADVANCED_FACE('',(#198),#169,.T.);
#1361=ADVANCED_FACE('',(#199),#1310,.T.);
#1362=ADVANCED_FACE('',(#200,#100),#1311,.T.);
#1363=ADVANCED_FACE('',(#201),#1312,.T.);
#1364=ADVANCED_FACE('',(#202),#170,.T.);
#1365=ADVANCED_FACE('',(#203),#1313,.T.);
#1366=ADVANCED_FACE('',(#204),#1314,.T.);
#1367=ADVANCED_FACE('',(#205),#171,.T.);
#1368=ADVANCED_FACE('',(#206),#1315,.T.);
#1369=ADVANCED_FACE('',(#207),#172,.T.);
#1370=ADVANCED_FACE('',(#208),#173,.T.);
#1371=ADVANCED_FACE('',(#209),#174,.T.);
#1372=ADVANCED_FACE('',(#210),#1316,.T.);
#1373=ADVANCED_FACE('',(#211),#175,.T.);
#1374=ADVANCED_FACE('',(#212),#1317,.T.);
#1375=ADVANCED_FACE('',(#213),#176,.T.);
#1376=ADVANCED_FACE('',(#214),#177,.T.);
#1377=ADVANCED_FACE('',(#215),#178,.T.);
#1378=ADVANCED_FACE('',(#216),#1318,.T.);
#1379=ADVANCED_FACE('',(#217),#179,.T.);
#1380=ADVANCED_FACE('',(#218),#1319,.T.);
#1381=ADVANCED_FACE('',(#219),#180,.T.);
#1382=ADVANCED_FACE('',(#220),#1320,.T.);
#1383=ADVANCED_FACE('',(#221),#181,.T.);
#1384=ADVANCED_FACE('',(#222,#101),#1321,.F.);
#1385=ADVANCED_FACE('',(#223),#182,.T.);
#1386=ADVANCED_FACE('',(#224),#1322,.T.);
#1387=ADVANCED_FACE('',(#225),#183,.T.);
#1388=ADVANCED_FACE('',(#226),#1323,.T.);
#1389=ADVANCED_FACE('',(#227),#1324,.T.);
#1390=ADVANCED_FACE('',(#228),#184,.T.);
#1391=ADVANCED_FACE('',(#229),#1325,.T.);
#1392=ADVANCED_FACE('',(#230),#185,.T.);
#1393=ADVANCED_FACE('',(#231),#1326,.T.);
#1394=ADVANCED_FACE('',(#232),#186,.T.);
#1395=ADVANCED_FACE('',(#233),#1327,.T.);
#1396=ADVANCED_FACE('',(#234),#1328,.T.);
#1397=ADVANCED_FACE('',(#235),#187,.F.);
#1443=CLOSED_SHELL('',(#1359,#1360,#1361,#1362,#1363,#1364,#1365,#1366,
#1367,#1368,#1369,#1370,#1371,#1372,#1373,#1374,#1375,#1376,#1377,#1378,
#1379,#1380,#1381,#1382,#1383,#1384,#1385,#1386,#1387,#1388,#1389,#1390,
#1391,#1392,#1393,#1394,#1395,#1396,#1397));
#1541=AXIS2_PLACEMENT_3D('',#2128,#1700,#1701);
#1542=AXIS2_PLACEMENT_3D('',#2129,#1702,#1703);
#1543=AXIS2_PLACEMENT_3D('',#2138,#1708,#1709);
#1544=AXIS2_PLACEMENT_3D('',#2142,#1711,#1712);
#1545=AXIS2_PLACEMENT_3D('',#2143,#1713,#1714);
#1546=AXIS2_PLACEMENT_3D('',#2144,#1715,#1716);
#1547=AXIS2_PLACEMENT_3D('',#2150,#1720,#1721);
#1548=AXIS2_PLACEMENT_3D('',#2152,#1722,#1723);
#1549=AXIS2_PLACEMENT_3D('',#2156,#1725,#1726);
#1550=AXIS2_PLACEMENT_3D('',#2160,#1728,#1729);
#1551=AXIS2_PLACEMENT_3D('',#2164,#1731,#1732);
#1552=AXIS2_PLACEMENT_3D('',#2168,#1734,#1735);
#1553=AXIS2_PLACEMENT_3D('',#2172,#1737,#1738);
#1554=AXIS2_PLACEMENT_3D('',#2176,#1740,#1741);
#1555=AXIS2_PLACEMENT_3D('',#2180,#1743,#1744);
#1556=AXIS2_PLACEMENT_3D('',#2184,#1746,#1747);
#1557=AXIS2_PLACEMENT_3D('',#2188,#1749,#1750);
#1558=AXIS2_PLACEMENT_3D('',#2192,#1752,#1753);
#1559=AXIS2_PLACEMENT_3D('',#2196,#1755,#1756);
#1560=AXIS2_PLACEMENT_3D('',#2200,#1758,#1759);
#1561=AXIS2_PLACEMENT_3D('',#2204,#1761,#1762);
#1562=AXIS2_PLACEMENT_3D('',#2208,#1764,#1765);
#1563=AXIS2_PLACEMENT_3D('',#2212,#1767,#1768);
#1564=AXIS2_PLACEMENT_3D('',#2215,#1770,#1771);
#1565=AXIS2_PLACEMENT_3D('',#2217,#1772,#1773);
#1566=AXIS2_PLACEMENT_3D('',#2218,#1774,#1775);
#1567=AXIS2_PLACEMENT_3D('',#2224,#1779,#1780);
#1568=AXIS2_PLACEMENT_3D('',#2227,#1782,#1783);
#1569=AXIS2_PLACEMENT_3D('',#2228,#1784,#1785);
#1570=AXIS2_PLACEMENT_3D('',#2232,#1788,#1789);
#1571=AXIS2_PLACEMENT_3D('',#2238,#1793,#1794);
#1572=AXIS2_PLACEMENT_3D('',#2241,#1796,#1797);
#1573=AXIS2_PLACEMENT_3D('',#2242,#1798,#1799);
#1574=AXIS2_PLACEMENT_3D('',#2246,#1802,#1803);
#1575=AXIS2_PLACEMENT_3D('',#2247,#1804,#1805);
#1576=AXIS2_PLACEMENT_3D('',#2248,#1806,#1807);
#1577=AXIS2_PLACEMENT_3D('',#2251,#1809,#1810);
#1578=AXIS2_PLACEMENT_3D('',#2252,#1811,#1812);
#1579=AXIS2_PLACEMENT_3D('',#2254,#1813,#1814);
#1580=AXIS2_PLACEMENT_3D('',#2256,#1816,#1817);
#1581=AXIS2_PLACEMENT_3D('',#2258,#1819,#1820);
#1582=AXIS2_PLACEMENT_3D('',#2262,#1822,#1823);
#1583=AXIS2_PLACEMENT_3D('',#2264,#1825,#1826);
#1584=AXIS2_PLACEMENT_3D('',#2268,#1829,#1830);
#1585=AXIS2_PLACEMENT_3D('',#2270,#1831,#1832);
#1586=AXIS2_PLACEMENT_3D('',#2272,#1834,#1835);
#1587=AXIS2_PLACEMENT_3D('',#2275,#1837,#1838);
#1588=AXIS2_PLACEMENT_3D('',#2276,#1839,#1840);
#1589=AXIS2_PLACEMENT_3D('',#2278,#1841,#1842);
#1590=AXIS2_PLACEMENT_3D('',#2280,#1844,#1845);
#1591=AXIS2_PLACEMENT_3D('',#2282,#1847,#1848);
#1592=AXIS2_PLACEMENT_3D('',#2286,#1850,#1851);
#1593=AXIS2_PLACEMENT_3D('',#2288,#1853,#1854);
#1594=AXIS2_PLACEMENT_3D('',#2292,#1857,#1858);
#1595=AXIS2_PLACEMENT_3D('',#2296,#1860,#1861);
#1596=AXIS2_PLACEMENT_3D('',#2298,#1863,#1864);
#1597=AXIS2_PLACEMENT_3D('',#2302,#1867,#1868);
#1598=AXIS2_PLACEMENT_3D('',#2304,#1869,#1870);
#1599=AXIS2_PLACEMENT_3D('',#2306,#1872,#1873);
#1600=AXIS2_PLACEMENT_3D('',#2310,#1875,#1876);
#1601=AXIS2_PLACEMENT_3D('',#2314,#1878,#1879);
#1602=AXIS2_PLACEMENT_3D('',#2318,#1881,#1882);
#1603=AXIS2_PLACEMENT_3D('',#2323,#1885,#1886);
#1604=AXIS2_PLACEMENT_3D('',#2326,#1888,#1889);
#1605=AXIS2_PLACEMENT_3D('',#2329,#1891,#1892);
#1606=AXIS2_PLACEMENT_3D('',#2330,#1893,#1894);
#1607=AXIS2_PLACEMENT_3D('',#2333,#1897,#1898);
#1608=AXIS2_PLACEMENT_3D('',#2334,#1899,#1900);
#1609=AXIS2_PLACEMENT_3D('',#2336,#1902,#1903);
#1610=AXIS2_PLACEMENT_3D('',#2337,#1904,#1905);
#1611=AXIS2_PLACEMENT_3D('',#2340,#1908,#1909);
#1612=AXIS2_PLACEMENT_3D('',#2342,#1911,#1912);
#1613=AXIS2_PLACEMENT_3D('',#2343,#1913,#1914);
#1614=AXIS2_PLACEMENT_3D('',#2346,#1917,#1918);
#1615=AXIS2_PLACEMENT_3D('',#2347,#1919,#1920);
#1616=AXIS2_PLACEMENT_3D('',#2349,#1922,#1923);
#1617=AXIS2_PLACEMENT_3D('',#2350,#1924,#1925);
#1618=AXIS2_PLACEMENT_3D('',#2351,#1926,#1927);
#1700=DIRECTION('axis',(0.,0.,1.));
#1701=DIRECTION('refdir',(1.,0.,0.));
#1702=DIRECTION('center_axis',(0.500081199337214,0.,0.865978518249416));
#1703=DIRECTION('ref_axis',(-0.865978518249416,0.,0.500081199337214));
#1704=DIRECTION('',(0.,-1.,0.));
#1705=DIRECTION('',(-0.865978518249416,0.,0.500081199337214));
#1706=DIRECTION('',(0.,-1.,0.));
#1707=DIRECTION('',(-0.865978518249416,0.,0.500081199337214));
#1708=DIRECTION('center_axis',(0.,-1.,0.));
#1709=DIRECTION('ref_axis',(-0.985840852699883,0.,-0.167683669890564));
#1710=DIRECTION('',(0.,1.,0.));
#1711=DIRECTION('center_axis',(0.,-1.,0.));
#1712=DIRECTION('ref_axis',(-0.985840852699883,0.,-0.167683669890564));
#1713=DIRECTION('center_axis',(0.,1.,0.));
#1714=DIRECTION('ref_axis',(-0.985840852699883,0.,-0.167683669890564));
#1715=DIRECTION('center_axis',(0.173740515882331,0.,0.984791466829878));
#1716=DIRECTION('ref_axis',(-0.984791466829877,0.,0.173740515882331));
#1717=DIRECTION('',(-0.984791466829877,0.,0.173740515882331));
#1718=DIRECTION('',(0.,-1.,0.));
#1719=DIRECTION('',(-0.984791466829877,0.,0.173740515882331));
#1720=DIRECTION('center_axis',(0.,1.,0.));
#1721=DIRECTION('ref_axis',(1.,0.,0.));
#1722=DIRECTION('center_axis',(0.,1.,0.));
#1723=DIRECTION('ref_axis',(-0.983738567360713,0.,0.179606322514249));
#1724=DIRECTION('',(-0.642715779886306,0.,0.766104709739562));
#1725=DIRECTION('center_axis',(0.,1.,0.));
#1726=DIRECTION('ref_axis',(-0.862982892362843,0.,0.505233141716833));
#1727=DIRECTION('',(-0.341932032994227,0.,0.939724685645979));
#1728=DIRECTION('center_axis',(0.,1.,0.));
#1729=DIRECTION('ref_axis',(-0.638138744274974,0.,0.769921387581329));
#1730=DIRECTION('',(9.37634563086646E-5,0.,0.999999995604207));
#1731=DIRECTION('center_axis',(0.,1.,0.));
#1732=DIRECTION('ref_axis',(-0.336325645702715,0.,0.941745751274011));
#1733=DIRECTION('',(0.342108250650212,0.,0.939660547664449));
#1734=DIRECTION('center_axis',(0.,1.,0.));
#1735=DIRECTION('ref_axis',(0.00605328937917962,0.,0.999981678676011));
#1736=DIRECTION('',(0.642859433835651,0.,0.765984169763649));
#1737=DIRECTION('center_axis',(0.,1.,0.));
#1738=DIRECTION('ref_axis',(0.347702108424909,0.,0.937605057471894));
#1739=DIRECTION('',(0.866072281705725,0.,0.499918796266994));
#1740=DIRECTION('center_axis',(0.,1.,0.));
#1741=DIRECTION('ref_axis',(0.647412921657998,0.,0.762139428759762));
#1742=DIRECTION('',(0.984824030536517,0.,0.173555837924887));
#1743=DIRECTION('center_axis',(0.,1.,0.));
#1744=DIRECTION('ref_axis',(0.869036181742023,0.,0.494748536959177));
#1745=DIRECTION('',(0.984791466829877,0.,-0.173740515882331));
#1746=DIRECTION('center_axis',(0.,1.,0.));
#1747=DIRECTION('ref_axis',(0.985840852699883,0.,0.167683669890565));
#1748=DIRECTION('',(0.865978518249416,0.,-0.500081199337213));
#1749=DIRECTION('center_axis',(0.,1.,0.));
#1750=DIRECTION('ref_axis',(0.983738567360713,0.,-0.179606322514249));
#1751=DIRECTION('',(0.642715779886305,0.,-0.766104709739562));
#1752=DIRECTION('center_axis',(0.,1.,0.));
#1753=DIRECTION('ref_axis',(0.862982892362843,0.,-0.505233141716833));
#1754=DIRECTION('',(0.341932032994227,0.,-0.93972468564598));
#1755=DIRECTION('center_axis',(0.,1.,0.));
#1756=DIRECTION('ref_axis',(0.638138744274974,0.,-0.769921387581329));
#1757=DIRECTION('',(-9.37634563085422E-5,0.,-0.999999995604207));
#1758=DIRECTION('center_axis',(0.,1.,0.));
#1759=DIRECTION('ref_axis',(0.336325645702715,0.,-0.941745751274011));
#1760=DIRECTION('',(-0.342108250650212,0.,-0.939660547664449));
#1761=DIRECTION('center_axis',(0.,1.,0.));
#1762=DIRECTION('ref_axis',(-0.00605328937917962,0.,-0.999981678676011));
#1763=DIRECTION('',(-0.642859433835651,0.,-0.765984169763649));
#1764=DIRECTION('center_axis',(0.,1.,0.));
#1765=DIRECTION('ref_axis',(-0.347702108424908,0.,-0.937605057471894));
#1766=DIRECTION('',(-0.866072281705724,0.,-0.499918796266994));
#1767=DIRECTION('center_axis',(0.,1.,0.));
#1768=DIRECTION('ref_axis',(-0.647412921657998,0.,-0.762139428759761));
#1769=DIRECTION('',(-0.984824030536517,0.,-0.173555837924887));
#1770=DIRECTION('center_axis',(0.,1.,0.));
#1771=DIRECTION('ref_axis',(-0.869036181742022,0.,-0.494748536959177));
#1772=DIRECTION('center_axis',(0.,-1.,0.));
#1773=DIRECTION('ref_axis',(1.,0.,0.));
#1774=DIRECTION('center_axis',(-0.173555837924887,0.,0.984824030536517));
#1775=DIRECTION('ref_axis',(-0.984824030536517,0.,-0.173555837924887));
#1776=DIRECTION('',(0.,-1.,0.));
#1777=DIRECTION('',(0.,-1.,0.));
#1778=DIRECTION('',(-0.984824030536517,0.,-0.173555837924887));
#1779=DIRECTION('center_axis',(0.,-1.,0.));
#1780=DIRECTION('ref_axis',(-0.647412921657998,0.,-0.762139428759761));
#1781=DIRECTION('',(0.,1.,0.));
#1782=DIRECTION('center_axis',(0.,-1.,0.));
#1783=DIRECTION('ref_axis',(-0.647412921657998,0.,-0.762139428759761));
#1784=DIRECTION('center_axis',(-0.499918796266994,0.,0.866072281705724));
#1785=DIRECTION('ref_axis',(-0.866072281705724,0.,-0.499918796266994));
#1786=DIRECTION('',(0.,-1.,0.));
#1787=DIRECTION('',(-0.866072281705724,0.,-0.499918796266994));
#1788=DIRECTION('center_axis',(-0.939660547664449,0.,0.342108250650212));
#1789=DIRECTION('ref_axis',(-0.342108250650212,0.,-0.939660547664449));
#1790=DIRECTION('',(0.,-1.,0.));
#1791=DIRECTION('',(0.,-1.,0.));
#1792=DIRECTION('',(-0.342108250650212,0.,-0.939660547664449));
#1793=DIRECTION('center_axis',(0.,-1.,0.));
#1794=DIRECTION('ref_axis',(0.336325645702715,0.,-0.941745751274011));
#1795=DIRECTION('',(0.,1.,0.));
#1796=DIRECTION('center_axis',(0.,-1.,0.));
#1797=DIRECTION('ref_axis',(0.336325645702715,0.,-0.941745751274011));
#1798=DIRECTION('center_axis',(-0.999999995604207,0.,9.37634563085422E-5));
#1799=DIRECTION('ref_axis',(-9.37634563085422E-5,0.,-0.999999995604207));
#1800=DIRECTION('',(0.,-1.,0.));
#1801=DIRECTION('',(-9.37634563085422E-5,0.,-0.999999995604207));
#1802=DIRECTION('center_axis',(0.,-1.,0.));
#1803=DIRECTION('ref_axis',(-0.869036181742022,0.,-0.494748536959177));
#1804=DIRECTION('center_axis',(0.,-1.,0.));
#1805=DIRECTION('ref_axis',(-0.869036181742022,0.,-0.494748536959177));
#1806=DIRECTION('center_axis',(0.,-1.,0.));
#1807=DIRECTION('ref_axis',(-0.347702108424908,0.,-0.937605057471894));
#1808=DIRECTION('',(0.,1.,0.));
#1809=DIRECTION('center_axis',(0.,-1.,0.));
#1810=DIRECTION('ref_axis',(-0.347702108424908,0.,-0.937605057471894));
#1811=DIRECTION('center_axis',(0.,-1.,0.));
#1812=DIRECTION('ref_axis',(-0.00605328937917962,0.,-0.999981678676011));
#1813=DIRECTION('center_axis',(0.,-1.,0.));
#1814=DIRECTION('ref_axis',(-0.00605328937917962,0.,-0.999981678676011));
#1815=DIRECTION('',(0.,-1.,0.));
#1816=DIRECTION('center_axis',(-0.765984169763649,0.,0.642859433835651));
#1817=DIRECTION('ref_axis',(-0.642859433835651,0.,-0.765984169763649));
#1818=DIRECTION('',(-0.642859433835651,0.,-0.765984169763649));
#1819=DIRECTION('center_axis',(0.,-1.,0.));
#1820=DIRECTION('ref_axis',(-0.862982892362843,0.,0.505233141716833));
#1821=DIRECTION('',(0.,1.,0.));
#1822=DIRECTION('center_axis',(0.,-1.,0.));
#1823=DIRECTION('ref_axis',(-0.862982892362843,0.,0.505233141716833));
#1824=DIRECTION('',(0.,-1.,0.));
#1825=DIRECTION('center_axis',(0.939724685645979,0.,0.341932032994227));
#1826=DIRECTION('ref_axis',(-0.341932032994227,0.,0.939724685645979));
#1827=DIRECTION('',(0.,-1.,0.));
#1828=DIRECTION('',(-0.341932032994227,0.,0.939724685645979));
#1829=DIRECTION('center_axis',(0.,-1.,0.));
#1830=DIRECTION('ref_axis',(-0.638138744274974,0.,0.769921387581329));
#1831=DIRECTION('center_axis',(0.,-1.,0.));
#1832=DIRECTION('ref_axis',(-0.638138744274974,0.,0.769921387581329));
#1833=DIRECTION('',(0.,-1.,0.));
#1834=DIRECTION('center_axis',(0.,-1.,0.));
#1835=DIRECTION('ref_axis',(0.638138744274974,0.,-0.769921387581329));
#1836=DIRECTION('',(0.,1.,0.));
#1837=DIRECTION('center_axis',(0.,-1.,0.));
#1838=DIRECTION('ref_axis',(0.638138744274974,0.,-0.769921387581329));
#1839=DIRECTION('center_axis',(0.,-1.,0.));
#1840=DIRECTION('ref_axis',(-0.983738567360713,0.,0.179606322514249));
#1841=DIRECTION('center_axis',(0.,-1.,0.));
#1842=DIRECTION('ref_axis',(-0.983738567360713,0.,0.179606322514249));
#1843=DIRECTION('',(0.,-1.,0.));
#1844=DIRECTION('center_axis',(0.766104709739562,0.,0.642715779886306));
#1845=DIRECTION('ref_axis',(-0.642715779886306,0.,0.766104709739562));
#1846=DIRECTION('',(-0.642715779886306,0.,0.766104709739562));
#1847=DIRECTION('center_axis',(0.,-1.,0.));
#1848=DIRECTION('ref_axis',(-0.336325645702715,0.,0.941745751274011));
#1849=DIRECTION('',(0.,1.,0.));
#1850=DIRECTION('center_axis',(0.,-1.,0.));
#1851=DIRECTION('ref_axis',(-0.336325645702715,0.,0.941745751274011));
#1852=DIRECTION('',(0.,-1.,0.));
#1853=DIRECTION('center_axis',(0.939660547664449,0.,-0.342108250650212));
#1854=DIRECTION('ref_axis',(0.342108250650212,0.,0.939660547664449));
#1855=DIRECTION('',(0.,-1.,0.));
#1856=DIRECTION('',(0.342108250650212,0.,0.939660547664449));
#1857=DIRECTION('center_axis',(0.,-1.,0.));
#1858=DIRECTION('ref_axis',(0.647412921657998,0.,0.762139428759762));
#1859=DIRECTION('',(0.,1.,0.));
#1860=DIRECTION('center_axis',(0.,-1.,0.));
#1861=DIRECTION('ref_axis',(0.647412921657998,0.,0.762139428759762));
#1862=DIRECTION('',(0.,-1.,0.));
#1863=DIRECTION('center_axis',(0.173555837924887,0.,-0.984824030536517));
#1864=DIRECTION('ref_axis',(0.984824030536517,0.,0.173555837924887));
#1865=DIRECTION('',(0.,-1.,0.));
#1866=DIRECTION('',(0.984824030536517,0.,0.173555837924887));
#1867=DIRECTION('center_axis',(0.,-1.,0.));
#1868=DIRECTION('ref_axis',(0.869036181742023,0.,0.494748536959177));
#1869=DIRECTION('center_axis',(0.,-1.,0.));
#1870=DIRECTION('ref_axis',(0.869036181742023,0.,0.494748536959177));
#1871=DIRECTION('',(0.,-1.,0.));
#1872=DIRECTION('center_axis',(0.,1.,0.));
#1873=DIRECTION('ref_axis',(1.,0.,0.));
#1874=DIRECTION('',(0.341932032994227,0.,-0.93972468564598));
#1875=DIRECTION('center_axis',(0.,-1.,0.));
#1876=DIRECTION('ref_axis',(0.862982892362843,0.,-0.505233141716833));
#1877=DIRECTION('',(0.642715779886305,0.,-0.766104709739562));
#1878=DIRECTION('center_axis',(0.,-1.,0.));
#1879=DIRECTION('ref_axis',(0.983738567360713,0.,-0.179606322514249));
#1880=DIRECTION('',(0.865978518249416,0.,-0.500081199337213));
#1881=DIRECTION('center_axis',(0.,-1.,0.));
#1882=DIRECTION('ref_axis',(0.985840852699883,0.,0.167683669890565));
#1883=DIRECTION('',(0.984791466829877,0.,-0.173740515882331));
#1884=DIRECTION('',(0.866072281705725,0.,0.499918796266994));
#1885=DIRECTION('center_axis',(0.,-1.,0.));
#1886=DIRECTION('ref_axis',(0.347702108424909,0.,0.937605057471894));
#1887=DIRECTION('',(0.642859433835651,0.,0.765984169763649));
#1888=DIRECTION('center_axis',(0.,-1.,0.));
#1889=DIRECTION('ref_axis',(0.00605328937917962,0.,0.999981678676011));
#1890=DIRECTION('',(9.37634563086646E-5,0.,0.999999995604207));
#1891=DIRECTION('center_axis',(0.,1.,0.));
#1892=DIRECTION('ref_axis',(1.,0.,0.));
#1893=DIRECTION('center_axis',(0.,-1.,0.));
#1894=DIRECTION('ref_axis',(0.347702108424909,0.,0.937605057471894));
#1895=DIRECTION('',(0.,1.,0.));
#1896=DIRECTION('',(0.,-1.,0.));
#1897=DIRECTION('center_axis',(0.499918796266994,0.,-0.866072281705725));
#1898=DIRECTION('ref_axis',(0.866072281705725,0.,0.499918796266994));
#1899=DIRECTION('center_axis',(0.,-1.,0.));
#1900=DIRECTION('ref_axis',(0.00605328937917962,0.,0.999981678676011));
#1901=DIRECTION('',(0.,-1.,0.));
#1902=DIRECTION('center_axis',(0.765984169763649,0.,-0.642859433835651));
#1903=DIRECTION('ref_axis',(0.642859433835651,0.,0.765984169763649));
#1904=DIRECTION('center_axis',(-0.500081199337213,0.,-0.865978518249416));
#1905=DIRECTION('ref_axis',(0.865978518249416,0.,-0.500081199337213));
#1906=DIRECTION('',(0.,-1.,0.));
#1907=DIRECTION('',(0.,-1.,0.));
#1908=DIRECTION('center_axis',(0.,-1.,0.));
#1909=DIRECTION('ref_axis',(0.985840852699883,0.,0.167683669890565));
#1910=DIRECTION('',(0.,1.,0.));
#1911=DIRECTION('center_axis',(-0.173740515882331,0.,-0.984791466829877));
#1912=DIRECTION('ref_axis',(0.984791466829877,0.,-0.173740515882331));
#1913=DIRECTION('center_axis',(0.,-1.,0.));
#1914=DIRECTION('ref_axis',(0.862982892362843,0.,-0.505233141716833));
#1915=DIRECTION('',(0.,1.,0.));
#1916=DIRECTION('',(0.,-1.,0.));
#1917=DIRECTION('center_axis',(-0.93972468564598,0.,-0.341932032994227));
#1918=DIRECTION('ref_axis',(0.341932032994227,0.,-0.93972468564598));
#1919=DIRECTION('center_axis',(0.,-1.,0.));
#1920=DIRECTION('ref_axis',(0.983738567360713,0.,-0.179606322514249));
#1921=DIRECTION('',(0.,-1.,0.));
#1922=DIRECTION('center_axis',(-0.766104709739562,0.,-0.642715779886305));
#1923=DIRECTION('ref_axis',(0.642715779886305,0.,-0.766104709739562));
#1924=DIRECTION('center_axis',(0.999999995604207,0.,-9.37634563086646E-5));
#1925=DIRECTION('ref_axis',(9.37634563086646E-5,0.,0.999999995604207));
#1926=DIRECTION('center_axis',(0.,-1.,0.));
#1927=DIRECTION('ref_axis',(1.,0.,0.));
#1928=DIRECTION('',(0.,1.,0.));
#2128=CARTESIAN_POINT('',(0.,0.,0.));
#2129=CARTESIAN_POINT('Origin',(-33.3281551220004,0.,66.411927135393));
#2130=CARTESIAN_POINT('',(-33.3724763544127,0.,66.4375215521063));
#2131=CARTESIAN_POINT('',(-33.3724763544127,-10.,66.4375215521063));
#2132=CARTESIAN_POINT('',(-33.3724763544127,0.,66.4375215521063));
#2133=CARTESIAN_POINT('',(-37.4153984446205,0.,68.7722091743641));
#2134=CARTESIAN_POINT('',(-33.3281551220004,0.,66.411927135393));
#2135=CARTESIAN_POINT('',(-37.4153984446205,-10.,68.7722091743641));
#2136=CARTESIAN_POINT('',(-37.4153984446205,0.,68.7722091743641));
#2137=CARTESIAN_POINT('',(-33.3281551220004,-10.,66.411927135393));
#2138=CARTESIAN_POINT('Origin',(-0.957463170361006,0.,59.9988083494084));
#2139=CARTESIAN_POINT('',(-37.9507118793475,-10.,53.8625915627806));
#2140=CARTESIAN_POINT('',(-37.9507118793475,0.,53.8625915627806));
#2141=CARTESIAN_POINT('',(-37.9507118793475,0.,53.8625915627806));
#2142=CARTESIAN_POINT('Origin',(-0.957463170361006,-10.,59.9988083494084));
#2143=CARTESIAN_POINT('Origin',(-0.957463170361006,0.,59.9988083494084));
#2144=CARTESIAN_POINT('Origin',(-37.900309738233,0.,53.8536994325238));
#2145=CARTESIAN_POINT('',(-42.5483261291134,0.,54.673719500509));
#2146=CARTESIAN_POINT('',(-37.900309738233,0.,53.8536994325238));
#2147=CARTESIAN_POINT('',(-42.5483261291134,-10.,54.673719500509));
#2148=CARTESIAN_POINT('',(-42.5483261291134,0.,54.673719500509));
#2149=CARTESIAN_POINT('',(-37.900309738233,-10.,53.8536994325238));
#2150=CARTESIAN_POINT('Origin',(-0.00360820116592997,0.,47.167824608198));
#2151=CARTESIAN_POINT('',(-27.7700567175474,0.,80.2648912227814));
#2152=CARTESIAN_POINT('Origin',(3.48851622115957,0.,59.5512429605134));
#2153=CARTESIAN_POINT('',(-24.7694628581521,0.,76.6882416995582));
#2154=CARTESIAN_POINT('',(-24.7365683291828,0.,76.6490320607774));
#2155=CARTESIAN_POINT('',(-14.7756715102625,0.,87.7655785767993));
#2156=CARTESIAN_POINT('Origin',(7.51329386908021,0.,57.6100545585387));
#2157=CARTESIAN_POINT('',(-13.1793217851717,0.,83.3783638708365));
#2158=CARTESIAN_POINT('',(-13.1618215253105,0.,83.3302682710978));
#2159=CARTESIAN_POINT('',(0.000442544535028677,0.,90.3695776431675));
#2160=CARTESIAN_POINT('Origin',(10.6314221896698,0.,54.4093791136522));
#2161=CARTESIAN_POINT('',(4.79886261666655E-6,0.,85.7009605963974));
#2162=CARTESIAN_POINT('',(0.,0.,85.6497800748447));
#2163=CARTESIAN_POINT('',(14.7760680196183,0.,87.7628077035488));
#2164=CARTESIAN_POINT('Origin',(12.4668088887924,0.,50.3352653214458));
#2165=CARTESIAN_POINT('',(13.1788956017712,0.,83.3758924332613));
#2166=CARTESIAN_POINT('',(13.1613863229985,0.,83.327800116138));
#2167=CARTESIAN_POINT('',(27.769046417685,0.,80.2596836844883));
#2168=CARTESIAN_POINT('Origin',(12.7980792431109,0.,45.8791114327754));
#2169=CARTESIAN_POINT('',(24.7677818930099,0.,76.6835969162539));
#2170=CARTESIAN_POINT('',(24.7348800117566,0.,76.644393446772));
#2171=CARTESIAN_POINT('',(37.4122327879896,0.,68.7651930770015));
#2172=CARTESIAN_POINT('Origin',(11.5852771588649,0.,41.5783953724418));
#2173=CARTESIAN_POINT('',(33.3688729521094,0.,66.4312636524891));
#2174=CARTESIAN_POINT('',(33.3245469208345,0.,66.4056775476497));
#2175=CARTESIAN_POINT('',(42.5425165359998,0.,54.6657410889655));
#2176=CARTESIAN_POINT('Origin',(8.97468446646684,0.,37.9518469691304));
#2177=CARTESIAN_POINT('',(37.9447502587574,0.,53.8554753419011));
#2178=CARTESIAN_POINT('',(37.8943464510154,0.,53.8465926635586));
#2179=CARTESIAN_POINT('',(42.5411097267815,0.,39.661929715887));
#2180=CARTESIAN_POINT('Origin',(5.28117717286475,0.,35.4368814824347));
#2181=CARTESIAN_POINT('',(37.9434954770157,0.,40.4730576536155));
#2182=CARTESIAN_POINT('',(37.8930933359011,0.,40.4819497838722));
#2183=CARTESIAN_POINT('',(37.4081820422886,0.,25.563440042032));
#2184=CARTESIAN_POINT('Origin',(0.950246768029155,0.,34.3368408669877));
#2185=CARTESIAN_POINT('',(33.3652599520808,0.,27.8981276642898));
#2186=CARTESIAN_POINT('',(33.3209387196686,0.,27.923722081003));
#2187=CARTESIAN_POINT('',(27.7628403152156,0.,14.0707579936147));
#2188=CARTESIAN_POINT('Origin',(-3.49573262349144,0.,34.7844062558827));
#2189=CARTESIAN_POINT('',(24.7622464558202,0.,17.6474075168379));
#2190=CARTESIAN_POINT('',(24.7293519268509,0.,17.6866171556187));
#2191=CARTESIAN_POINT('',(14.7684551079306,0.,6.57007063959682));
#2192=CARTESIAN_POINT('Origin',(-7.52051027141208,0.,36.7255946578574));
#2193=CARTESIAN_POINT('',(13.1721053828398,0.,10.9572853455596));
#2194=CARTESIAN_POINT('',(13.1546051229786,0.,11.0053809452983));
#2195=CARTESIAN_POINT('',(-0.00765894686688301,0.,3.9660715732286));
#2196=CARTESIAN_POINT('Origin',(-10.6386385920017,0.,39.9262701027439));
#2197=CARTESIAN_POINT('',(-0.00722120119447005,0.,8.63468861999872));
#2198=CARTESIAN_POINT('',(-0.00721640233185491,0.,8.68586914155136));
#2199=CARTESIAN_POINT('',(-14.7832844219502,0.,6.57284151284728));
#2200=CARTESIAN_POINT('Origin',(-12.4740252911242,0.,44.0003838949503));
#2201=CARTESIAN_POINT('',(-13.1861120041031,0.,10.9597567831348));
#2202=CARTESIAN_POINT('',(-13.1686027253304,0.,11.0078491002581));
#2203=CARTESIAN_POINT('',(-27.7762628200168,0.,14.0759655319078));
#2204=CARTESIAN_POINT('Origin',(-12.8052956454428,0.,48.4565377836207));
#2205=CARTESIAN_POINT('',(-24.7749982953418,0.,17.6520523001422));
#2206=CARTESIAN_POINT('',(-24.7420964140884,0.,17.6912557696241));
#2207=CARTESIAN_POINT('',(-37.4194491903214,0.,25.5704561393946));
#2208=CARTESIAN_POINT('Origin',(-11.5924935611967,0.,52.7572538439543));
#2209=CARTESIAN_POINT('',(-33.3760893544412,0.,27.904385563907));
#2210=CARTESIAN_POINT('',(-33.3317633231664,0.,27.9299716687463));
#2211=CARTESIAN_POINT('',(-42.5497329383317,0.,39.6699081274306));
#2212=CARTESIAN_POINT('Origin',(-8.9819008687987,0.,56.3838022472657));
#2213=CARTESIAN_POINT('',(-37.9519666610893,0.,40.480173874495));
#2214=CARTESIAN_POINT('',(-37.9015628533472,0.,40.4890565528375));
#2215=CARTESIAN_POINT('Origin',(-5.28839357519661,0.,58.8987677339614));
#2216=CARTESIAN_POINT('',(-14.4855638369713,0.,47.167824608198));
#2217=CARTESIAN_POINT('Origin',(-0.00360820116592981,0.,47.167824608198));
#2218=CARTESIAN_POINT('Origin',(-37.9015628533472,0.,40.4890565528375));
#2219=CARTESIAN_POINT('',(-37.9519666610893,-10.,40.480173874495));
#2220=CARTESIAN_POINT('',(-37.9519666610893,0.,40.480173874495));
#2221=CARTESIAN_POINT('',(-42.5497329383317,-10.,39.6699081274306));
#2222=CARTESIAN_POINT('',(-42.5497329383317,0.,39.6699081274306));
#2223=CARTESIAN_POINT('',(-37.9015628533472,-10.,40.4890565528375));
#2224=CARTESIAN_POINT('Origin',(-8.9819008687987,0.,56.3838022472657));
#2225=CARTESIAN_POINT('',(-33.3760893544412,-10.,27.904385563907));
#2226=CARTESIAN_POINT('',(-33.3760893544412,0.,27.904385563907));
#2227=CARTESIAN_POINT('Origin',(-8.9819008687987,-10.,56.3838022472657));
#2228=CARTESIAN_POINT('Origin',(-33.3317633231664,0.,27.9299716687463));
#2229=CARTESIAN_POINT('',(-37.4194491903214,-10.,25.5704561393946));
#2230=CARTESIAN_POINT('',(-37.4194491903214,0.,25.5704561393946));
#2231=CARTESIAN_POINT('',(-33.3317633231664,-10.,27.9299716687463));
#2232=CARTESIAN_POINT('Origin',(-13.1686027253304,0.,11.0078491002581));
#2233=CARTESIAN_POINT('',(-13.1861120041031,-10.,10.9597567831348));
#2234=CARTESIAN_POINT('',(-13.1861120041031,0.,10.9597567831348));
#2235=CARTESIAN_POINT('',(-14.7832844219502,-10.,6.57284151284728));
#2236=CARTESIAN_POINT('',(-14.7832844219502,0.,6.57284151284728));
#2237=CARTESIAN_POINT('',(-13.1686027253304,-10.,11.0078491002581));
#2238=CARTESIAN_POINT('Origin',(-12.4740252911242,0.,44.0003838949503));
#2239=CARTESIAN_POINT('',(-0.00722120119447227,-10.,8.63468861999872));
#2240=CARTESIAN_POINT('',(-0.00722120119447227,0.,8.63468861999872));
#2241=CARTESIAN_POINT('Origin',(-12.4740252911242,-10.,44.0003838949503));
#2242=CARTESIAN_POINT('Origin',(-0.00721640233185491,0.,8.68586914155136));
#2243=CARTESIAN_POINT('',(-0.00765894686688301,-10.,3.9660715732286));
#2244=CARTESIAN_POINT('',(-0.00765894686688301,0.,3.9660715732286));
#2245=CARTESIAN_POINT('',(-0.00721640233185491,-10.,8.68586914155136));
#2246=CARTESIAN_POINT('Origin',(-5.28839357519661,0.,58.8987677339614));
#2247=CARTESIAN_POINT('Origin',(-5.28839357519661,-10.,58.8987677339614));
#2248=CARTESIAN_POINT('Origin',(-11.5924935611967,0.,52.7572538439543));
#2249=CARTESIAN_POINT('',(-24.7749982953418,-10.,17.6520523001422));
#2250=CARTESIAN_POINT('',(-24.7749982953418,0.,17.6520523001422));
#2251=CARTESIAN_POINT('Origin',(-11.5924935611967,-10.,52.7572538439543));
#2252=CARTESIAN_POINT('Origin',(-12.8052956454428,0.,48.4565377836207));
#2253=CARTESIAN_POINT('',(-27.7762628200168,-10.,14.0759655319078));
#2254=CARTESIAN_POINT('Origin',(-12.8052956454428,-10.,48.4565377836207));
#2255=CARTESIAN_POINT('',(-27.7762628200168,0.,14.0759655319078));
#2256=CARTESIAN_POINT('Origin',(-24.7420964140884,0.,17.6912557696241));
#2257=CARTESIAN_POINT('',(-24.7420964140884,-10.,17.6912557696241));
#2258=CARTESIAN_POINT('Origin',(7.51329386908021,0.,57.6100545585387));
#2259=CARTESIAN_POINT('',(-24.7694628581521,-10.,76.6882416995582));
#2260=CARTESIAN_POINT('',(-24.7694628581521,0.,76.6882416995582));
#2261=CARTESIAN_POINT('',(-14.7756715102625,-10.,87.7655785767993));
#2262=CARTESIAN_POINT('Origin',(7.51329386908021,-10.,57.6100545585387));
#2263=CARTESIAN_POINT('',(-14.7756715102625,0.,87.7655785767993));
#2264=CARTESIAN_POINT('Origin',(-13.1618215253105,0.,83.3302682710978));
#2265=CARTESIAN_POINT('',(-13.1793217851717,-10.,83.3783638708365));
#2266=CARTESIAN_POINT('',(-13.1793217851717,0.,83.3783638708365));
#2267=CARTESIAN_POINT('',(-13.1618215253105,-10.,83.3302682710978));
#2268=CARTESIAN_POINT('Origin',(10.6314221896698,0.,54.4093791136522));
#2269=CARTESIAN_POINT('',(0.000442544535028677,-10.,90.3695776431675));
#2270=CARTESIAN_POINT('Origin',(10.6314221896698,-10.,54.4093791136522));
#2271=CARTESIAN_POINT('',(0.000442544535028677,0.,90.3695776431675));
#2272=CARTESIAN_POINT('Origin',(-10.6386385920017,0.,39.9262701027439));
#2273=CARTESIAN_POINT('',(13.1721053828398,-10.,10.9572853455596));
#2274=CARTESIAN_POINT('',(13.1721053828398,0.,10.9572853455596));
#2275=CARTESIAN_POINT('Origin',(-10.6386385920017,-10.,39.9262701027439));
#2276=CARTESIAN_POINT('Origin',(3.48851622115957,0.,59.5512429605134));
#2277=CARTESIAN_POINT('',(-27.7700567175474,-10.,80.2648912227814));
#2278=CARTESIAN_POINT('Origin',(3.48851622115957,-10.,59.5512429605134));
#2279=CARTESIAN_POINT('',(-27.7700567175474,0.,80.2648912227814));
#2280=CARTESIAN_POINT('Origin',(-24.7365683291828,0.,76.6490320607774));
#2281=CARTESIAN_POINT('',(-24.7365683291828,-10.,76.6490320607774));
#2282=CARTESIAN_POINT('Origin',(12.4668088887924,0.,50.3352653214458));
#2283=CARTESIAN_POINT('',(4.79886261666655E-6,-10.,85.7009605963974));
#2284=CARTESIAN_POINT('',(4.798862618887E-6,0.,85.7009605963974));
#2285=CARTESIAN_POINT('',(14.7760680196183,-10.,87.7628077035488));
#2286=CARTESIAN_POINT('Origin',(12.4668088887924,-10.,50.3352653214458));
#2287=CARTESIAN_POINT('',(14.7760680196183,0.,87.7628077035488));
#2288=CARTESIAN_POINT('Origin',(13.1613863229985,0.,83.327800116138));
#2289=CARTESIAN_POINT('',(13.1788956017712,-10.,83.3758924332613));
#2290=CARTESIAN_POINT('',(13.1788956017712,0.,83.3758924332613));
#2291=CARTESIAN_POINT('',(13.1613863229985,-10.,83.327800116138));
#2292=CARTESIAN_POINT('Origin',(8.97468446646684,0.,37.9518469691304));
#2293=CARTESIAN_POINT('',(33.3688729521094,-10.,66.4312636524891));
#2294=CARTESIAN_POINT('',(33.3688729521094,0.,66.4312636524891));
#2295=CARTESIAN_POINT('',(42.5425165359998,-10.,54.6657410889655));
#2296=CARTESIAN_POINT('Origin',(8.97468446646684,-10.,37.9518469691304));
#2297=CARTESIAN_POINT('',(42.5425165359998,0.,54.6657410889655));
#2298=CARTESIAN_POINT('Origin',(37.8943464510154,0.,53.8465926635586));
#2299=CARTESIAN_POINT('',(37.9447502587574,-10.,53.8554753419011));
#2300=CARTESIAN_POINT('',(37.9447502587574,0.,53.8554753419011));
#2301=CARTESIAN_POINT('',(37.8943464510154,-10.,53.8465926635586));
#2302=CARTESIAN_POINT('Origin',(5.28117717286475,0.,35.4368814824347));
#2303=CARTESIAN_POINT('',(42.5411097267815,-10.,39.661929715887));
#2304=CARTESIAN_POINT('Origin',(5.28117717286475,-10.,35.4368814824347));
#2305=CARTESIAN_POINT('',(42.5411097267815,0.,39.661929715887));
#2306=CARTESIAN_POINT('Origin',(-0.00360820116592997,-10.,47.167824608198));
#2307=CARTESIAN_POINT('',(14.7684551079306,-10.,6.57007063959682));
#2308=CARTESIAN_POINT('',(13.1546051229786,-10.,11.0053809452983));
#2309=CARTESIAN_POINT('',(24.7622464558202,-10.,17.6474075168379));
#2310=CARTESIAN_POINT('Origin',(-7.52051027141208,-10.,36.7255946578574));
#2311=CARTESIAN_POINT('',(27.7628403152156,-10.,14.0707579936147));
#2312=CARTESIAN_POINT('',(24.7293519268509,-10.,17.6866171556187));
#2313=CARTESIAN_POINT('',(33.3652599520808,-10.,27.8981276642898));
#2314=CARTESIAN_POINT('Origin',(-3.49573262349144,-10.,34.7844062558827));
#2315=CARTESIAN_POINT('',(37.4081820422886,-10.,25.563440042032));
#2316=CARTESIAN_POINT('',(33.3209387196686,-10.,27.923722081003));
#2317=CARTESIAN_POINT('',(37.9434954770157,-10.,40.4730576536155));
#2318=CARTESIAN_POINT('Origin',(0.950246768029155,-10.,34.3368408669877));
#2319=CARTESIAN_POINT('',(37.8930933359011,-10.,40.4819497838722));
#2320=CARTESIAN_POINT('',(37.4122327879896,-10.,68.7651930770015));
#2321=CARTESIAN_POINT('',(33.3245469208345,-10.,66.4056775476497));
#2322=CARTESIAN_POINT('',(24.7677818930099,-10.,76.6835969162539));
#2323=CARTESIAN_POINT('Origin',(11.5852771588649,-10.,41.5783953724418));
#2324=CARTESIAN_POINT('',(27.769046417685,-10.,80.2596836844883));
#2325=CARTESIAN_POINT('',(24.7348800117566,-10.,76.644393446772));
#2326=CARTESIAN_POINT('Origin',(12.7980792431109,-10.,45.8791114327754));
#2327=CARTESIAN_POINT('',(0.,-10.,85.6497800748447));
#2328=CARTESIAN_POINT('',(-14.4855638369713,-10.,47.167824608198));
#2329=CARTESIAN_POINT('Origin',(-0.00360820116592981,-10.,47.167824608198));
#2330=CARTESIAN_POINT('Origin',(11.5852771588649,0.,41.5783953724418));
#2331=CARTESIAN_POINT('',(24.7677818930099,0.,76.6835969162539));
#2332=CARTESIAN_POINT('',(37.4122327879896,0.,68.7651930770015));
#2333=CARTESIAN_POINT('Origin',(33.3245469208345,0.,66.4056775476497));
#2334=CARTESIAN_POINT('Origin',(12.7980792431109,0.,45.8791114327754));
#2335=CARTESIAN_POINT('',(27.769046417685,0.,80.2596836844883));
#2336=CARTESIAN_POINT('Origin',(24.7348800117566,0.,76.644393446772));
#2337=CARTESIAN_POINT('Origin',(33.3209387196686,0.,27.923722081003));
#2338=CARTESIAN_POINT('',(33.3652599520808,0.,27.8981276642898));
#2339=CARTESIAN_POINT('',(37.4081820422886,0.,25.563440042032));
#2340=CARTESIAN_POINT('Origin',(0.950246768029155,0.,34.3368408669877));
#2341=CARTESIAN_POINT('',(37.9434954770157,0.,40.4730576536155));
#2342=CARTESIAN_POINT('Origin',(37.8930933359011,0.,40.4819497838722));
#2343=CARTESIAN_POINT('Origin',(-7.52051027141208,0.,36.7255946578574));
#2344=CARTESIAN_POINT('',(24.7622464558202,0.,17.6474075168379));
#2345=CARTESIAN_POINT('',(14.7684551079306,0.,6.57007063959682));
#2346=CARTESIAN_POINT('Origin',(13.1546051229786,0.,11.0053809452983));
#2347=CARTESIAN_POINT('Origin',(-3.49573262349144,0.,34.7844062558827));
#2348=CARTESIAN_POINT('',(27.7628403152156,0.,14.0707579936147));
#2349=CARTESIAN_POINT('Origin',(24.7293519268509,0.,17.6866171556187));
#2350=CARTESIAN_POINT('Origin',(0.,0.,85.6497800748447));
#2351=CARTESIAN_POINT('Origin',(-0.00360820116592981,0.,47.167824608198));
#2352=CARTESIAN_POINT('',(-14.4855638369713,0.,47.167824608198));
#4061=UNCERTAINTY_MEASURE_WITH_UNIT(LENGTH_MEASURE(0.01),#4080,
'DISTANCE_ACCURACY_VALUE',
'Maximum model space distance between geometric entities at asserted c
onnectivities');
#4069=UNCERTAINTY_MEASURE_WITH_UNIT(LENGTH_MEASURE(0.01),#4080,
'DISTANCE_ACCURACY_VALUE',
'Maximum model space distance between geometric entities at asserted c
onnectivities');
#4071=(
GEOMETRIC_REPRESENTATION_CONTEXT(3)
GLOBAL_UNCERTAINTY_ASSIGNED_CONTEXT((#4061))
GLOBAL_UNIT_ASSIGNED_CONTEXT((#4080,#4082,#4083))
REPRESENTATION_CONTEXT('','3D')
);
#4079=(
GEOMETRIC_REPRESENTATION_CONTEXT(3)
GLOBAL_UNCERTAINTY_ASSIGNED_CONTEXT((#4069))
GLOBAL_UNIT_ASSIGNED_CONTEXT((#4080,#4082,#4083))
REPRESENTATION_CONTEXT('','3D')
);
#4080=(
LENGTH_UNIT()
NAMED_UNIT(*)
SI_UNIT(.MILLI.,.METRE.)
);
#4082=(
NAMED_UNIT(*)
PLANE_ANGLE_UNIT()
SI_UNIT($,.RADIAN.)
);
#4083=(
NAMED_UNIT(*)
SI_UNIT($,.STERADIAN.)
SOLID_ANGLE_UNIT()
);
#4085=SHAPE_DEFINITION_REPRESENTATION(#4094,#4111);
#4094=PRODUCT_DEFINITION_SHAPE('',$,#4121);
#4111=SHAPE_REPRESENTATION('',(#1541),#4071);
#4119=PRODUCT_DEFINITION_CONTEXT('part definition',#4148,'design');
#4121=PRODUCT_DEFINITION('Wheel','Wheel',#4130,#4119);
#4130=PRODUCT_DEFINITION_FORMATION('',$,#4151);
#4148=APPLICATION_CONTEXT(
'Core Data for Automotive Mechanical Design Process');
#4149=PRODUCT_CONTEXT('part definition',#4148,'mechanical');
#4151=PRODUCT('Wheel','Wheel',$,(#4149));
#4160=PRESENTATION_STYLE_ASSIGNMENT((#4164));
#4164=SURFACE_STYLE_USAGE(.BOTH.,#4168);
#4168=SURFACE_SIDE_STYLE('',(#4172));
#4172=SURFACE_STYLE_FILL_AREA(#4176);
#4176=FILL_AREA_STYLE('Stainless Steel - Polished',(#4180));
#4180=FILL_AREA_STYLE_COLOUR('Stainless Steel - Polished',#4184);
#4184=COLOUR_RGB('Stainless Steel - Polished', 0.09019608, 0.27058824, 0.51372549);
ENDSEC;
END-ISO-10303-21;
